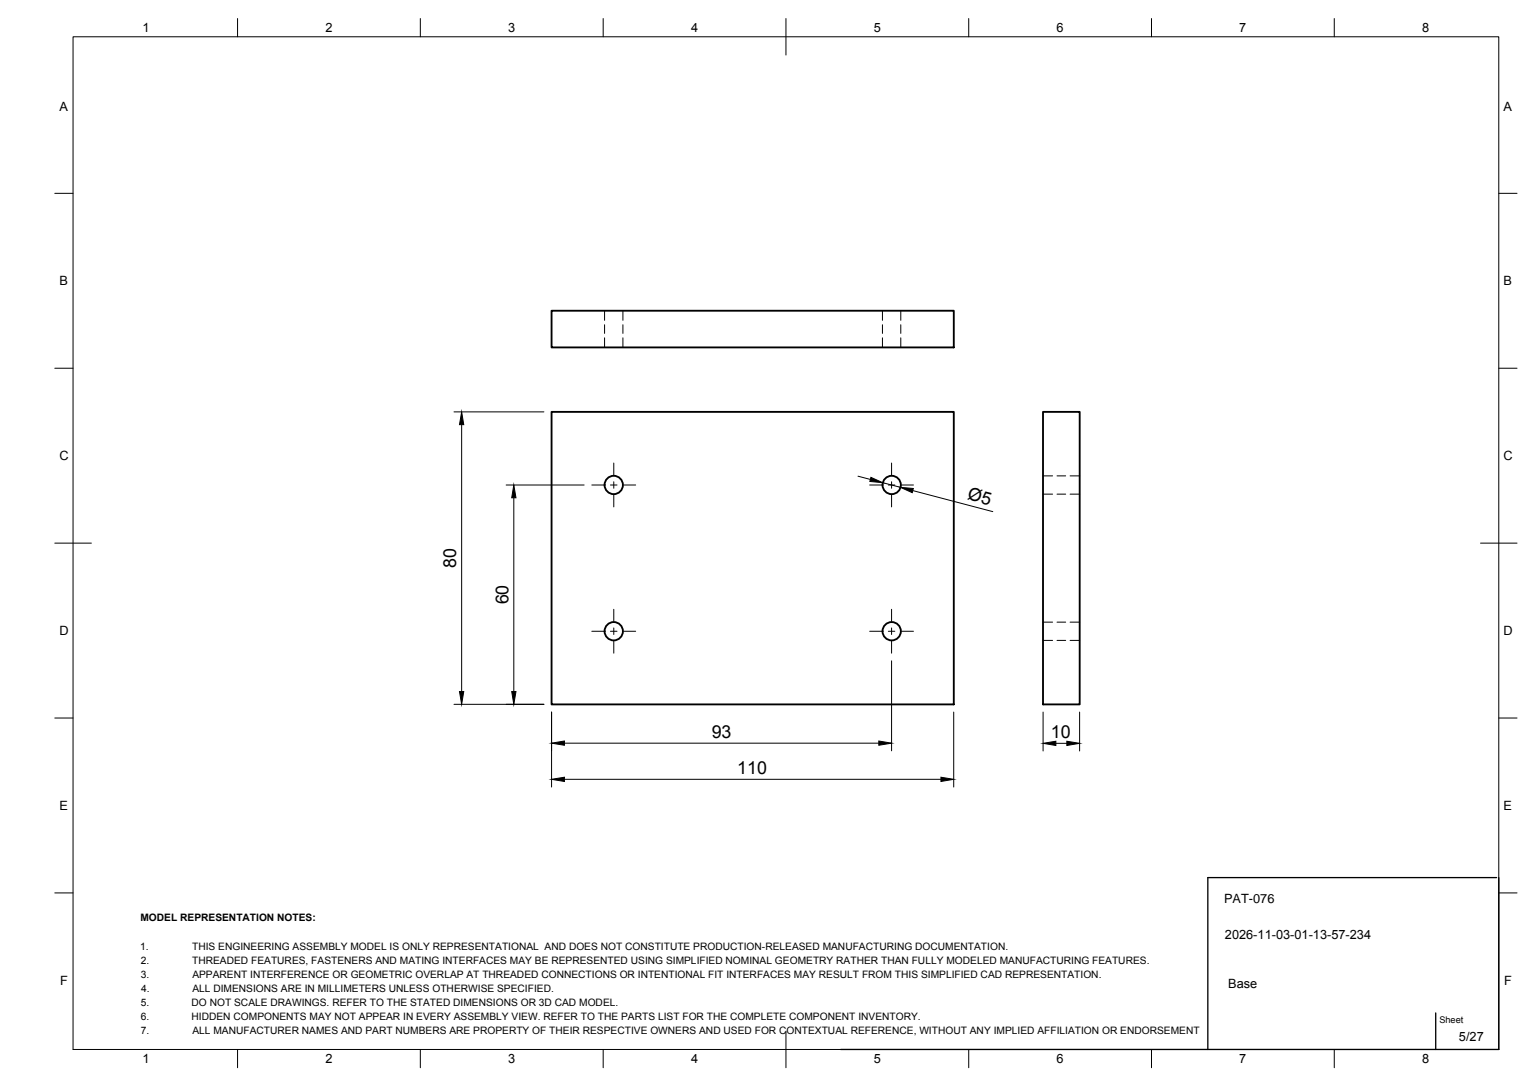
ISO-10303-21;
HEADER;
/* Generated by software containing ST-Developer
 * from STEP Tools, Inc. (www.steptools.com) 
 */

FILE_DESCRIPTION(
/* description */ ('Overhung pulley bearing cartridge'),
/* implementation_level */ '2;1');

FILE_NAME(
/* name */ 'Base.step',
/* time_stamp */ '2026-10-28T03:22:33-07:00',
/* author */ (''),
/* organization */ (''),
/* preprocessor_version */ 'ST-DEVELOPER v20.2',
/* originating_system */ 'Autodesk Translation Framework v15.17.0.0',
/* authorisation */ '');

FILE_SCHEMA (('AUTOMOTIVE_DESIGN { 1 0 10303 214 3 1 1 }'));
ENDSEC;

DATA;
#10=MECHANICAL_DESIGN_GEOMETRIC_PRESENTATION_REPRESENTATION('',(#283),#10963);
#239=SHAPE_REPRESENTATION_RELATIONSHIP('SRR','None',#11059,#261);
#261=ADVANCED_BREP_SHAPE_REPRESENTATION('',(#313),#10939);
#283=STYLED_ITEM('',(#11232),#313);
#313=MANIFOLD_SOLID_BREP('Body1',#5650);
#341=FACE_BOUND('',#915,.T.);
#342=FACE_BOUND('',#916,.T.);
#343=FACE_BOUND('',#917,.T.);
#344=FACE_BOUND('',#918,.T.);
#345=FACE_BOUND('',#920,.T.);
#346=FACE_BOUND('',#921,.T.);
#347=FACE_BOUND('',#922,.T.);
#348=FACE_BOUND('',#923,.T.);
#434=PLANE('',#5940);
#435=PLANE('',#5941);
#436=PLANE('',#5942);
#437=PLANE('',#5943);
#438=PLANE('',#5944);
#439=PLANE('',#5945);
#577=FACE_OUTER_BOUND('',#906,.T.);
#578=FACE_OUTER_BOUND('',#907,.T.);
#579=FACE_OUTER_BOUND('',#908,.T.);
#580=FACE_OUTER_BOUND('',#909,.T.);
#581=FACE_OUTER_BOUND('',#910,.T.);
#582=FACE_OUTER_BOUND('',#911,.T.);
#583=FACE_OUTER_BOUND('',#912,.T.);
#584=FACE_OUTER_BOUND('',#913,.T.);
#585=FACE_OUTER_BOUND('',#914,.T.);
#586=FACE_OUTER_BOUND('',#919,.T.);
#906=EDGE_LOOP('',(#3653,#3654,#3655,#3656));
#907=EDGE_LOOP('',(#3657,#3658,#3659,#3660));
#908=EDGE_LOOP('',(#3661,#3662,#3663,#3664));
#909=EDGE_LOOP('',(#3665,#3666,#3667,#3668));
#910=EDGE_LOOP('',(#3669,#3670,#3671,#3672));
#911=EDGE_LOOP('',(#3673,#3674,#3675,#3676));
#912=EDGE_LOOP('',(#3677,#3678,#3679,#3680));
#913=EDGE_LOOP('',(#3681,#3682,#3683,#3684));
#914=EDGE_LOOP('',(#3685,#3686,#3687,#3688));
#915=EDGE_LOOP('',(#3689));
#916=EDGE_LOOP('',(#3690));
#917=EDGE_LOOP('',(#3691));
#918=EDGE_LOOP('',(#3692));
#919=EDGE_LOOP('',(#3693,#3694,#3695,#3696));
#920=EDGE_LOOP('',(#3697));
#921=EDGE_LOOP('',(#3698));
#922=EDGE_LOOP('',(#3699));
#923=EDGE_LOOP('',(#3700));
#1328=LINE('',#8563,#1670);
#1329=LINE('',#8569,#1671);
#1330=LINE('',#8575,#1672);
#1331=LINE('',#8581,#1673);
#1332=LINE('',#8586,#1674);
#1333=LINE('',#8588,#1675);
#1334=LINE('',#8590,#1676);
#1335=LINE('',#8591,#1677);
#1336=LINE('',#8594,#1678);
#1337=LINE('',#8596,#1679);
#1338=LINE('',#8597,#1680);
#1339=LINE('',#8600,#1681);
#1340=LINE('',#8602,#1682);
#1341=LINE('',#8603,#1683);
#1342=LINE('',#8605,#1684);
#1343=LINE('',#8606,#1685);
#1670=VECTOR('',#6698,0.25);
#1671=VECTOR('',#6705,0.25);
#1672=VECTOR('',#6712,0.25);
#1673=VECTOR('',#6719,0.25);
#1674=VECTOR('',#6724,1.);
#1675=VECTOR('',#6725,1.);
#1676=VECTOR('',#6726,1.);
#1677=VECTOR('',#6727,1.);
#1678=VECTOR('',#6730,1.);
#1679=VECTOR('',#6731,1.);
#1680=VECTOR('',#6732,1.);
#1681=VECTOR('',#6735,1.);
#1682=VECTOR('',#6736,1.);
#1683=VECTOR('',#6737,1.);
#1684=VECTOR('',#6740,1.);
#1685=VECTOR('',#6741,1.);
#2012=CIRCLE('',#5929,0.25);
#2013=CIRCLE('',#5930,0.25);
#2014=CIRCLE('',#5932,0.25);
#2015=CIRCLE('',#5933,0.25);
#2016=CIRCLE('',#5935,0.25);
#2017=CIRCLE('',#5936,0.25);
#2018=CIRCLE('',#5938,0.25);
#2019=CIRCLE('',#5939,0.25);
#2383=VERTEX_POINT('',#8560);
#2384=VERTEX_POINT('',#8562);
#2385=VERTEX_POINT('',#8566);
#2386=VERTEX_POINT('',#8568);
#2387=VERTEX_POINT('',#8572);
#2388=VERTEX_POINT('',#8574);
#2389=VERTEX_POINT('',#8578);
#2390=VERTEX_POINT('',#8580);
#2391=VERTEX_POINT('',#8584);
#2392=VERTEX_POINT('',#8585);
#2393=VERTEX_POINT('',#8587);
#2394=VERTEX_POINT('',#8589);
#2395=VERTEX_POINT('',#8593);
#2396=VERTEX_POINT('',#8595);
#2397=VERTEX_POINT('',#8599);
#2398=VERTEX_POINT('',#8601);
#2896=EDGE_CURVE('',#2383,#2383,#2012,.T.);
#2897=EDGE_CURVE('',#2383,#2384,#1328,.T.);
#2898=EDGE_CURVE('',#2384,#2384,#2013,.T.);
#2899=EDGE_CURVE('',#2385,#2385,#2014,.T.);
#2900=EDGE_CURVE('',#2385,#2386,#1329,.T.);
#2901=EDGE_CURVE('',#2386,#2386,#2015,.T.);
#2902=EDGE_CURVE('',#2387,#2387,#2016,.T.);
#2903=EDGE_CURVE('',#2387,#2388,#1330,.T.);
#2904=EDGE_CURVE('',#2388,#2388,#2017,.T.);
#2905=EDGE_CURVE('',#2389,#2389,#2018,.T.);
#2906=EDGE_CURVE('',#2389,#2390,#1331,.T.);
#2907=EDGE_CURVE('',#2390,#2390,#2019,.T.);
#2908=EDGE_CURVE('',#2391,#2392,#1332,.T.);
#2909=EDGE_CURVE('',#2392,#2393,#1333,.T.);
#2910=EDGE_CURVE('',#2394,#2393,#1334,.T.);
#2911=EDGE_CURVE('',#2391,#2394,#1335,.T.);
#2912=EDGE_CURVE('',#2395,#2391,#1336,.T.);
#2913=EDGE_CURVE('',#2396,#2394,#1337,.T.);
#2914=EDGE_CURVE('',#2395,#2396,#1338,.T.);
#2915=EDGE_CURVE('',#2397,#2395,#1339,.T.);
#2916=EDGE_CURVE('',#2398,#2396,#1340,.T.);
#2917=EDGE_CURVE('',#2397,#2398,#1341,.T.);
#2918=EDGE_CURVE('',#2392,#2397,#1342,.T.);
#2919=EDGE_CURVE('',#2393,#2398,#1343,.T.);
#3653=ORIENTED_EDGE('',*,*,#2896,.F.);
#3654=ORIENTED_EDGE('',*,*,#2897,.T.);
#3655=ORIENTED_EDGE('',*,*,#2898,.F.);
#3656=ORIENTED_EDGE('',*,*,#2897,.F.);
#3657=ORIENTED_EDGE('',*,*,#2899,.F.);
#3658=ORIENTED_EDGE('',*,*,#2900,.T.);
#3659=ORIENTED_EDGE('',*,*,#2901,.F.);
#3660=ORIENTED_EDGE('',*,*,#2900,.F.);
#3661=ORIENTED_EDGE('',*,*,#2902,.F.);
#3662=ORIENTED_EDGE('',*,*,#2903,.T.);
#3663=ORIENTED_EDGE('',*,*,#2904,.F.);
#3664=ORIENTED_EDGE('',*,*,#2903,.F.);
#3665=ORIENTED_EDGE('',*,*,#2905,.F.);
#3666=ORIENTED_EDGE('',*,*,#2906,.T.);
#3667=ORIENTED_EDGE('',*,*,#2907,.F.);
#3668=ORIENTED_EDGE('',*,*,#2906,.F.);
#3669=ORIENTED_EDGE('',*,*,#2908,.T.);
#3670=ORIENTED_EDGE('',*,*,#2909,.T.);
#3671=ORIENTED_EDGE('',*,*,#2910,.F.);
#3672=ORIENTED_EDGE('',*,*,#2911,.F.);
#3673=ORIENTED_EDGE('',*,*,#2912,.T.);
#3674=ORIENTED_EDGE('',*,*,#2911,.T.);
#3675=ORIENTED_EDGE('',*,*,#2913,.F.);
#3676=ORIENTED_EDGE('',*,*,#2914,.F.);
#3677=ORIENTED_EDGE('',*,*,#2915,.T.);
#3678=ORIENTED_EDGE('',*,*,#2914,.T.);
#3679=ORIENTED_EDGE('',*,*,#2916,.F.);
#3680=ORIENTED_EDGE('',*,*,#2917,.F.);
#3681=ORIENTED_EDGE('',*,*,#2918,.T.);
#3682=ORIENTED_EDGE('',*,*,#2917,.T.);
#3683=ORIENTED_EDGE('',*,*,#2919,.F.);
#3684=ORIENTED_EDGE('',*,*,#2909,.F.);
#3685=ORIENTED_EDGE('',*,*,#2919,.T.);
#3686=ORIENTED_EDGE('',*,*,#2916,.T.);
#3687=ORIENTED_EDGE('',*,*,#2913,.T.);
#3688=ORIENTED_EDGE('',*,*,#2910,.T.);
#3689=ORIENTED_EDGE('',*,*,#2898,.T.);
#3690=ORIENTED_EDGE('',*,*,#2901,.T.);
#3691=ORIENTED_EDGE('',*,*,#2904,.T.);
#3692=ORIENTED_EDGE('',*,*,#2907,.T.);
#3693=ORIENTED_EDGE('',*,*,#2918,.F.);
#3694=ORIENTED_EDGE('',*,*,#2908,.F.);
#3695=ORIENTED_EDGE('',*,*,#2912,.F.);
#3696=ORIENTED_EDGE('',*,*,#2915,.F.);
#3697=ORIENTED_EDGE('',*,*,#2896,.T.);
#3698=ORIENTED_EDGE('',*,*,#2899,.T.);
#3699=ORIENTED_EDGE('',*,*,#2902,.T.);
#3700=ORIENTED_EDGE('',*,*,#2905,.T.);
#5167=CYLINDRICAL_SURFACE('',#5928,0.25);
#5168=CYLINDRICAL_SURFACE('',#5931,0.25);
#5169=CYLINDRICAL_SURFACE('',#5934,0.25);
#5170=CYLINDRICAL_SURFACE('',#5937,0.25);
#5321=ADVANCED_FACE('',(#577),#5167,.F.);
#5322=ADVANCED_FACE('',(#578),#5168,.F.);
#5323=ADVANCED_FACE('',(#579),#5169,.F.);
#5324=ADVANCED_FACE('',(#580),#5170,.F.);
#5325=ADVANCED_FACE('',(#581),#434,.T.);
#5326=ADVANCED_FACE('',(#582),#435,.T.);
#5327=ADVANCED_FACE('',(#583),#436,.T.);
#5328=ADVANCED_FACE('',(#584),#437,.T.);
#5329=ADVANCED_FACE('',(#585,#341,#342,#343,#344),#438,.T.);
#5330=ADVANCED_FACE('',(#586,#345,#346,#347,#348),#439,.F.);
#5650=CLOSED_SHELL('',(#5321,#5322,#5323,#5324,#5325,#5326,#5327,#5328,
#5329,#5330));
#5927=AXIS2_PLACEMENT_3D('',#8558,#6692,#6693);
#5928=AXIS2_PLACEMENT_3D('',#8559,#6694,#6695);
#5929=AXIS2_PLACEMENT_3D('',#8561,#6696,#6697);
#5930=AXIS2_PLACEMENT_3D('',#8564,#6699,#6700);
#5931=AXIS2_PLACEMENT_3D('',#8565,#6701,#6702);
#5932=AXIS2_PLACEMENT_3D('',#8567,#6703,#6704);
#5933=AXIS2_PLACEMENT_3D('',#8570,#6706,#6707);
#5934=AXIS2_PLACEMENT_3D('',#8571,#6708,#6709);
#5935=AXIS2_PLACEMENT_3D('',#8573,#6710,#6711);
#5936=AXIS2_PLACEMENT_3D('',#8576,#6713,#6714);
#5937=AXIS2_PLACEMENT_3D('',#8577,#6715,#6716);
#5938=AXIS2_PLACEMENT_3D('',#8579,#6717,#6718);
#5939=AXIS2_PLACEMENT_3D('',#8582,#6720,#6721);
#5940=AXIS2_PLACEMENT_3D('',#8583,#6722,#6723);
#5941=AXIS2_PLACEMENT_3D('',#8592,#6728,#6729);
#5942=AXIS2_PLACEMENT_3D('',#8598,#6733,#6734);
#5943=AXIS2_PLACEMENT_3D('',#8604,#6738,#6739);
#5944=AXIS2_PLACEMENT_3D('',#8607,#6742,#6743);
#5945=AXIS2_PLACEMENT_3D('',#8608,#6744,#6745);
#6692=DIRECTION('axis',(0.,0.,1.));
#6693=DIRECTION('refdir',(1.,0.,0.));
#6694=DIRECTION('center_axis',(0.,0.,1.));
#6695=DIRECTION('ref_axis',(1.,0.,0.));
#6696=DIRECTION('center_axis',(0.,0.,1.));
#6697=DIRECTION('ref_axis',(1.,0.,0.));
#6698=DIRECTION('',(0.,0.,1.));
#6699=DIRECTION('center_axis',(0.,0.,-1.));
#6700=DIRECTION('ref_axis',(1.,0.,0.));
#6701=DIRECTION('center_axis',(0.,0.,1.));
#6702=DIRECTION('ref_axis',(1.,0.,0.));
#6703=DIRECTION('center_axis',(0.,0.,1.));
#6704=DIRECTION('ref_axis',(1.,0.,0.));
#6705=DIRECTION('',(0.,0.,1.));
#6706=DIRECTION('center_axis',(0.,0.,-1.));
#6707=DIRECTION('ref_axis',(1.,0.,0.));
#6708=DIRECTION('center_axis',(0.,0.,1.));
#6709=DIRECTION('ref_axis',(1.,0.,0.));
#6710=DIRECTION('center_axis',(0.,0.,1.));
#6711=DIRECTION('ref_axis',(1.,0.,0.));
#6712=DIRECTION('',(0.,0.,1.));
#6713=DIRECTION('center_axis',(0.,0.,-1.));
#6714=DIRECTION('ref_axis',(1.,0.,0.));
#6715=DIRECTION('center_axis',(0.,0.,1.));
#6716=DIRECTION('ref_axis',(1.,0.,0.));
#6717=DIRECTION('center_axis',(0.,0.,1.));
#6718=DIRECTION('ref_axis',(1.,0.,0.));
#6719=DIRECTION('',(0.,0.,1.));
#6720=DIRECTION('center_axis',(0.,0.,-1.));
#6721=DIRECTION('ref_axis',(1.,0.,0.));
#6722=DIRECTION('center_axis',(0.,1.,0.));
#6723=DIRECTION('ref_axis',(-1.,0.,0.));
#6724=DIRECTION('',(-1.,0.,0.));
#6725=DIRECTION('',(0.,0.,1.));
#6726=DIRECTION('',(-1.,0.,0.));
#6727=DIRECTION('',(0.,0.,1.));
#6728=DIRECTION('center_axis',(1.,0.,0.));
#6729=DIRECTION('ref_axis',(0.,1.,0.));
#6730=DIRECTION('',(0.,1.,0.));
#6731=DIRECTION('',(0.,1.,0.));
#6732=DIRECTION('',(0.,0.,1.));
#6733=DIRECTION('center_axis',(0.,-1.,0.));
#6734=DIRECTION('ref_axis',(1.,0.,0.));
#6735=DIRECTION('',(1.,0.,0.));
#6736=DIRECTION('',(1.,0.,0.));
#6737=DIRECTION('',(0.,0.,1.));
#6738=DIRECTION('center_axis',(-1.,0.,0.));
#6739=DIRECTION('ref_axis',(0.,-1.,0.));
#6740=DIRECTION('',(0.,-1.,0.));
#6741=DIRECTION('',(0.,-1.,0.));
#6742=DIRECTION('center_axis',(0.,0.,1.));
#6743=DIRECTION('ref_axis',(1.,0.,0.));
#6744=DIRECTION('center_axis',(0.,0.,1.));
#6745=DIRECTION('ref_axis',(1.,0.,0.));
#8558=CARTESIAN_POINT('',(0.,0.,0.));
#8559=CARTESIAN_POINT('Origin',(3.8,1.,-0.1));
#8560=CARTESIAN_POINT('',(3.55,1.,0.));
#8561=CARTESIAN_POINT('Origin',(3.8,1.,0.));
#8562=CARTESIAN_POINT('',(3.55,1.,1.));
#8563=CARTESIAN_POINT('',(3.55,1.,-0.1));
#8564=CARTESIAN_POINT('Origin',(3.8,1.,1.));
#8565=CARTESIAN_POINT('Origin',(-3.8,5.,-0.1));
#8566=CARTESIAN_POINT('',(-4.05,5.,0.));
#8567=CARTESIAN_POINT('Origin',(-3.8,5.,0.));
#8568=CARTESIAN_POINT('',(-4.05,5.,1.));
#8569=CARTESIAN_POINT('',(-4.05,5.,-0.1));
#8570=CARTESIAN_POINT('Origin',(-3.8,5.,1.));
#8571=CARTESIAN_POINT('Origin',(-3.8,1.,-0.1));
#8572=CARTESIAN_POINT('',(-4.05,1.,0.));
#8573=CARTESIAN_POINT('Origin',(-3.8,1.,0.));
#8574=CARTESIAN_POINT('',(-4.05,1.,1.));
#8575=CARTESIAN_POINT('',(-4.05,1.,-0.1));
#8576=CARTESIAN_POINT('Origin',(-3.8,1.,1.));
#8577=CARTESIAN_POINT('Origin',(3.8,5.,-0.1));
#8578=CARTESIAN_POINT('',(3.55,5.,0.));
#8579=CARTESIAN_POINT('Origin',(3.8,5.,0.));
#8580=CARTESIAN_POINT('',(3.55,5.,1.));
#8581=CARTESIAN_POINT('',(3.55,5.,-0.1));
#8582=CARTESIAN_POINT('Origin',(3.8,5.,1.));
#8583=CARTESIAN_POINT('Origin',(5.5,7.,0.));
#8584=CARTESIAN_POINT('',(5.5,7.,0.));
#8585=CARTESIAN_POINT('',(-5.5,7.,0.));
#8586=CARTESIAN_POINT('',(5.5,7.,0.));
#8587=CARTESIAN_POINT('',(-5.5,7.,1.));
#8588=CARTESIAN_POINT('',(-5.5,7.,0.));
#8589=CARTESIAN_POINT('',(5.5,7.,1.));
#8590=CARTESIAN_POINT('',(5.5,7.,1.));
#8591=CARTESIAN_POINT('',(5.5,7.,0.));
#8592=CARTESIAN_POINT('Origin',(5.5,-1.,0.));
#8593=CARTESIAN_POINT('',(5.5,-1.,0.));
#8594=CARTESIAN_POINT('',(5.5,-1.,0.));
#8595=CARTESIAN_POINT('',(5.5,-1.,1.));
#8596=CARTESIAN_POINT('',(5.5,-1.,1.));
#8597=CARTESIAN_POINT('',(5.5,-1.,0.));
#8598=CARTESIAN_POINT('Origin',(-5.5,-1.,0.));
#8599=CARTESIAN_POINT('',(-5.5,-1.,0.));
#8600=CARTESIAN_POINT('',(-5.5,-1.,0.));
#8601=CARTESIAN_POINT('',(-5.5,-1.,1.));
#8602=CARTESIAN_POINT('',(-5.5,-1.,1.));
#8603=CARTESIAN_POINT('',(-5.5,-1.,0.));
#8604=CARTESIAN_POINT('Origin',(-5.5,7.,0.));
#8605=CARTESIAN_POINT('',(-5.5,7.,0.));
#8606=CARTESIAN_POINT('',(-5.5,7.,1.));
#8607=CARTESIAN_POINT('Origin',(0.,3.,1.));
#8608=CARTESIAN_POINT('Origin',(0.,3.,0.));
#10912=UNCERTAINTY_MEASURE_WITH_UNIT(LENGTH_MEASURE(0.001),#10964,
'DISTANCE_ACCURACY_VALUE',
'Maximum model space distance between geometric entities at asserted c
onnectivities');
#10936=UNCERTAINTY_MEASURE_WITH_UNIT(LENGTH_MEASURE(0.001),#10964,
'DISTANCE_ACCURACY_VALUE',
'Maximum model space distance between geometric entities at asserted c
onnectivities');
#10939=(
GEOMETRIC_REPRESENTATION_CONTEXT(3)
GLOBAL_UNCERTAINTY_ASSIGNED_CONTEXT((#10912))
GLOBAL_UNIT_ASSIGNED_CONTEXT((#10964,#10966,#10967))
REPRESENTATION_CONTEXT('','3D')
);
#10963=(
GEOMETRIC_REPRESENTATION_CONTEXT(3)
GLOBAL_UNCERTAINTY_ASSIGNED_CONTEXT((#10936))
GLOBAL_UNIT_ASSIGNED_CONTEXT((#10964,#10966,#10967))
REPRESENTATION_CONTEXT('','3D')
);
#10964=(
LENGTH_UNIT()
NAMED_UNIT(*)
SI_UNIT(.CENTI.,.METRE.)
);
#10966=(
NAMED_UNIT(*)
PLANE_ANGLE_UNIT()
SI_UNIT($,.RADIAN.)
);
#10967=(
NAMED_UNIT(*)
SI_UNIT($,.STERADIAN.)
SOLID_ANGLE_UNIT()
);
#10970=SHAPE_DEFINITION_REPRESENTATION(#10996,#11059);
#10996=PRODUCT_DEFINITION_SHAPE('',$,#11086);
#11059=SHAPE_REPRESENTATION('',(#5927),#10939);
#11083=PRODUCT_DEFINITION_CONTEXT('part definition',#11163,'design');
#11086=PRODUCT_DEFINITION('Base','Base',#11112,#11083);
#11112=PRODUCT_DEFINITION_FORMATION('',$,#11167);
#11163=APPLICATION_CONTEXT(
'Core Data for Automotive Mechanical Design Process');
#11164=PRODUCT_CONTEXT('part definition',#11163,'mechanical');
#11167=PRODUCT('Base','Base','Base',(#11164));
#11226=COLOUR_RGB('Dark Blue',0.08,0.2,0.34);
#11227=FILL_AREA_STYLE_COLOUR('',#11226);
#11228=FILL_AREA_STYLE('',(#11227));
#11229=SURFACE_STYLE_FILL_AREA(#11228);
#11230=SURFACE_SIDE_STYLE('',(#11229));
#11231=SURFACE_STYLE_USAGE(.BOTH.,#11230);
#11232=PRESENTATION_STYLE_ASSIGNMENT((#11231));
ENDSEC;
END-ISO-10303-21;
